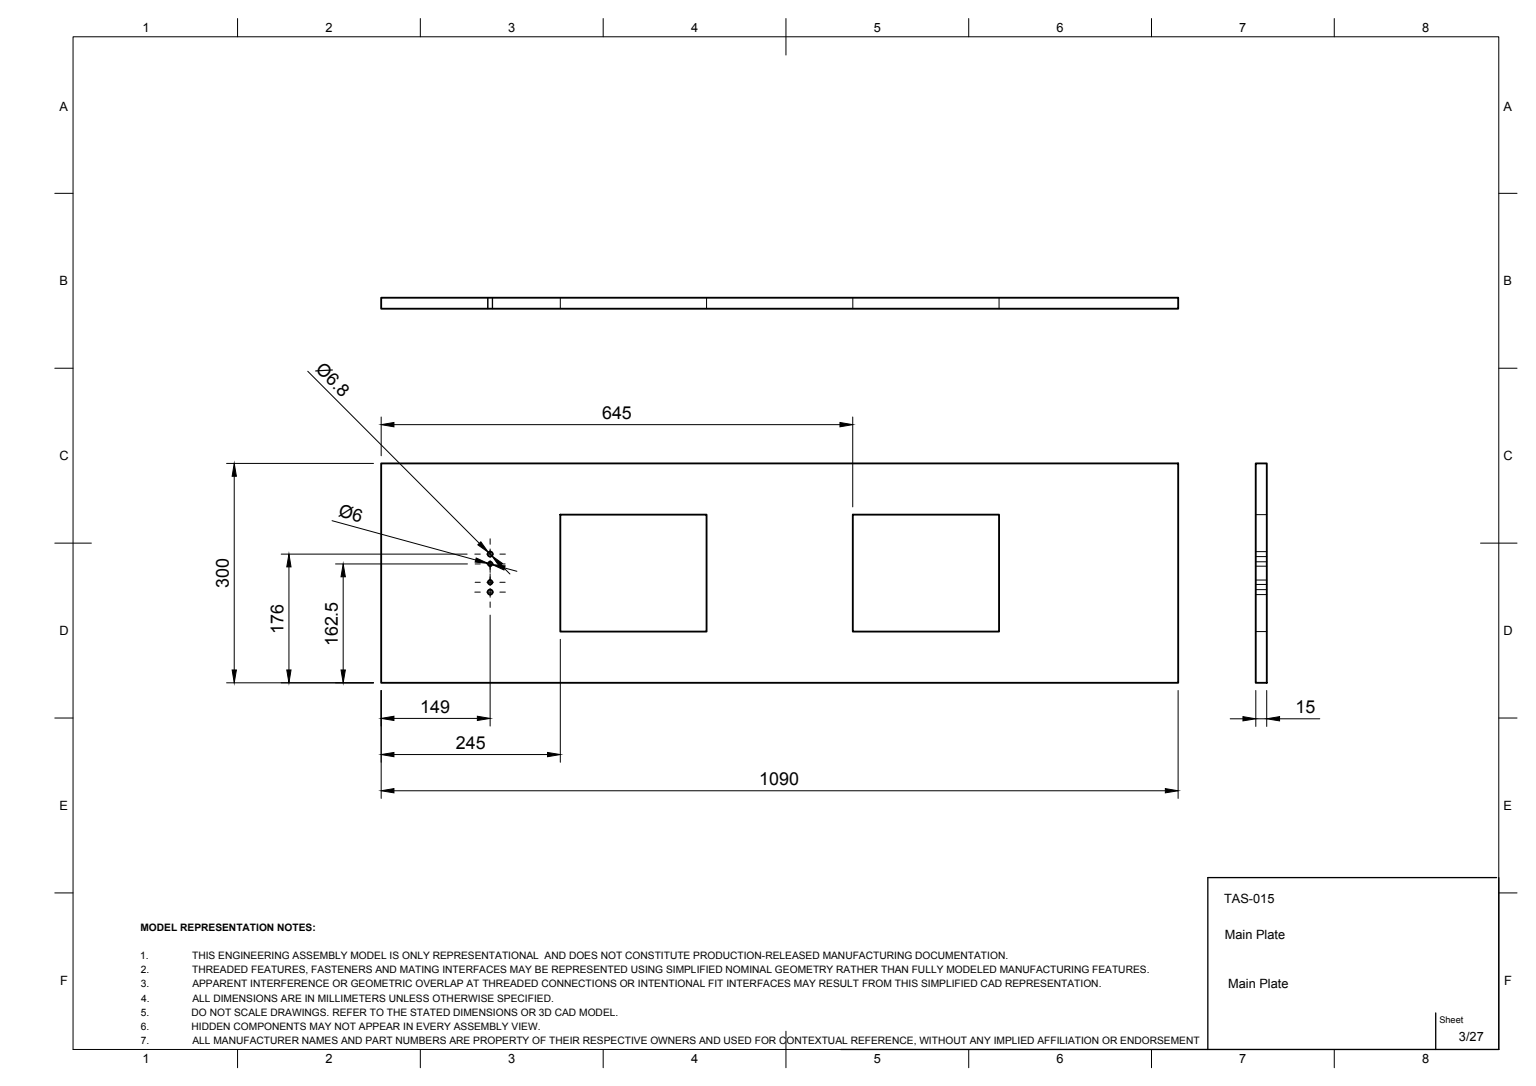
ISO-10303-21;
HEADER;
/* Generated by software containing ST-Developer
 * from STEP Tools, Inc. (www.steptools.com) 
 */

FILE_DESCRIPTION(
/* description */ ('STEP AP214'),
/* implementation_level */ '2;1');

FILE_NAME(
/* name */ 'Main Plate.step',
/* time_stamp */ '2026-11-15T14:49:54-08:00',
/* author */ (''),
/* organization */ (''),
/* preprocessor_version */ 'ST-DEVELOPER v20.2',
/* originating_system */ 'Autodesk Translation Framework v15.17.0.0',
/* authorisation */ '');

FILE_SCHEMA (('AUTOMOTIVE_DESIGN { 1 0 10303 214 3 1 1 }'));
ENDSEC;

DATA;
#10=MECHANICAL_DESIGN_GEOMETRIC_PRESENTATION_REPRESENTATION('',(#1098),#66721);
#1036=SHAPE_REPRESENTATION_RELATIONSHIP('SRR','None',#66891,#1067);
#1067=ADVANCED_BREP_SHAPE_REPRESENTATION('',(#1133),#66682);
#1098=STYLED_ITEM('',(#67095),#1133);
#1133=MANIFOLD_SOLID_BREP('Body1',#25664);
#1168=FACE_BOUND('',#3720,.T.);
#1169=FACE_BOUND('',#3721,.T.);
#1170=FACE_BOUND('',#3722,.T.);
#1171=FACE_BOUND('',#3723,.T.);
#1172=FACE_BOUND('',#3724,.T.);
#1173=FACE_BOUND('',#3725,.T.);
#1174=FACE_BOUND('',#3727,.T.);
#1175=FACE_BOUND('',#3728,.T.);
#1176=FACE_BOUND('',#3729,.T.);
#1177=FACE_BOUND('',#3730,.T.);
#1178=FACE_BOUND('',#3731,.T.);
#1179=FACE_BOUND('',#3732,.T.);
#1498=PLANE('',#26055);
#1499=PLANE('',#26056);
#1500=PLANE('',#26057);
#1501=PLANE('',#26058);
#1502=PLANE('',#26059);
#1503=PLANE('',#26060);
#1504=PLANE('',#26061);
#1505=PLANE('',#26062);
#1506=PLANE('',#26063);
#1507=PLANE('',#26064);
#1508=PLANE('',#26065);
#1509=PLANE('',#26066);
#1510=PLANE('',#26067);
#1511=PLANE('',#26068);
#2269=FACE_OUTER_BOUND('',#3711,.T.);
#2270=FACE_OUTER_BOUND('',#3712,.T.);
#2271=FACE_OUTER_BOUND('',#3713,.T.);
#2272=FACE_OUTER_BOUND('',#3714,.T.);
#2273=FACE_OUTER_BOUND('',#3715,.T.);
#2274=FACE_OUTER_BOUND('',#3716,.T.);
#2275=FACE_OUTER_BOUND('',#3717,.T.);
#2276=FACE_OUTER_BOUND('',#3718,.T.);
#2277=FACE_OUTER_BOUND('',#3719,.T.);
#2278=FACE_OUTER_BOUND('',#3726,.T.);
#2279=FACE_OUTER_BOUND('',#3733,.T.);
#2280=FACE_OUTER_BOUND('',#3734,.T.);
#2281=FACE_OUTER_BOUND('',#3735,.T.);
#2282=FACE_OUTER_BOUND('',#3736,.T.);
#2283=FACE_OUTER_BOUND('',#3737,.T.);
#2284=FACE_OUTER_BOUND('',#3738,.T.);
#2285=FACE_OUTER_BOUND('',#3739,.T.);
#2286=FACE_OUTER_BOUND('',#3740,.T.);
#3711=EDGE_LOOP('',(#16594,#16595,#16596,#16597));
#3712=EDGE_LOOP('',(#16598,#16599,#16600,#16601));
#3713=EDGE_LOOP('',(#16602,#16603,#16604,#16605));
#3714=EDGE_LOOP('',(#16606,#16607,#16608,#16609));
#3715=EDGE_LOOP('',(#16610,#16611,#16612,#16613));
#3716=EDGE_LOOP('',(#16614,#16615,#16616,#16617));
#3717=EDGE_LOOP('',(#16618,#16619,#16620,#16621));
#3718=EDGE_LOOP('',(#16622,#16623,#16624,#16625));
#3719=EDGE_LOOP('',(#16626,#16627,#16628,#16629));
#3720=EDGE_LOOP('',(#16630));
#3721=EDGE_LOOP('',(#16631));
#3722=EDGE_LOOP('',(#16632));
#3723=EDGE_LOOP('',(#16633));
#3724=EDGE_LOOP('',(#16634,#16635,#16636,#16637));
#3725=EDGE_LOOP('',(#16638,#16639,#16640,#16641));
#3726=EDGE_LOOP('',(#16642,#16643,#16644,#16645));
#3727=EDGE_LOOP('',(#16646));
#3728=EDGE_LOOP('',(#16647));
#3729=EDGE_LOOP('',(#16648));
#3730=EDGE_LOOP('',(#16649));
#3731=EDGE_LOOP('',(#16650,#16651,#16652,#16653));
#3732=EDGE_LOOP('',(#16654,#16655,#16656,#16657));
#3733=EDGE_LOOP('',(#16658,#16659,#16660,#16661));
#3734=EDGE_LOOP('',(#16662,#16663,#16664,#16665));
#3735=EDGE_LOOP('',(#16666,#16667,#16668,#16669));
#3736=EDGE_LOOP('',(#16670,#16671,#16672,#16673));
#3737=EDGE_LOOP('',(#16674,#16675,#16676,#16677));
#3738=EDGE_LOOP('',(#16678,#16679,#16680,#16681));
#3739=EDGE_LOOP('',(#16682,#16683,#16684,#16685));
#3740=EDGE_LOOP('',(#16686,#16687,#16688,#16689));
#5483=LINE('',#36181,#7472);
#5484=LINE('',#36187,#7473);
#5485=LINE('',#36193,#7474);
#5486=LINE('',#36199,#7475);
#5487=LINE('',#36204,#7476);
#5488=LINE('',#36206,#7477);
#5489=LINE('',#36208,#7478);
#5490=LINE('',#36209,#7479);
#5491=LINE('',#36212,#7480);
#5492=LINE('',#36214,#7481);
#5493=LINE('',#36215,#7482);
#5494=LINE('',#36218,#7483);
#5495=LINE('',#36220,#7484);
#5496=LINE('',#36221,#7485);
#5497=LINE('',#36223,#7486);
#5498=LINE('',#36224,#7487);
#5499=LINE('',#36228,#7488);
#5500=LINE('',#36230,#7489);
#5501=LINE('',#36232,#7490);
#5502=LINE('',#36233,#7491);
#5503=LINE('',#36236,#7492);
#5504=LINE('',#36238,#7493);
#5505=LINE('',#36240,#7494);
#5506=LINE('',#36241,#7495);
#5507=LINE('',#36245,#7496);
#5508=LINE('',#36247,#7497);
#5509=LINE('',#36249,#7498);
#5510=LINE('',#36250,#7499);
#5511=LINE('',#36253,#7500);
#5512=LINE('',#36255,#7501);
#5513=LINE('',#36257,#7502);
#5514=LINE('',#36258,#7503);
#5515=LINE('',#36260,#7504);
#5516=LINE('',#36261,#7505);
#5517=LINE('',#36263,#7506);
#5518=LINE('',#36265,#7507);
#5519=LINE('',#36268,#7508);
#5520=LINE('',#36269,#7509);
#5521=LINE('',#36271,#7510);
#5522=LINE('',#36273,#7511);
#7472=VECTOR('',#28764,3.4);
#7473=VECTOR('',#28771,3.4);
#7474=VECTOR('',#28778,2.99999999999999);
#7475=VECTOR('',#28785,2.99999999999999);
#7476=VECTOR('',#28790,1000.);
#7477=VECTOR('',#28791,1000.);
#7478=VECTOR('',#28792,1000.);
#7479=VECTOR('',#28793,1000.);
#7480=VECTOR('',#28796,1000.);
#7481=VECTOR('',#28797,1000.);
#7482=VECTOR('',#28798,1000.);
#7483=VECTOR('',#28801,1000.);
#7484=VECTOR('',#28802,1000.);
#7485=VECTOR('',#28803,1000.);
#7486=VECTOR('',#28806,1000.);
#7487=VECTOR('',#28807,1000.);
#7488=VECTOR('',#28810,1000.);
#7489=VECTOR('',#28811,1000.);
#7490=VECTOR('',#28812,1000.);
#7491=VECTOR('',#28813,1000.);
#7492=VECTOR('',#28814,1000.);
#7493=VECTOR('',#28815,1000.);
#7494=VECTOR('',#28816,1000.);
#7495=VECTOR('',#28817,1000.);
#7496=VECTOR('',#28820,1000.);
#7497=VECTOR('',#28821,1000.);
#7498=VECTOR('',#28822,1000.);
#7499=VECTOR('',#28823,1000.);
#7500=VECTOR('',#28824,1000.);
#7501=VECTOR('',#28825,1000.);
#7502=VECTOR('',#28826,1000.);
#7503=VECTOR('',#28827,1000.);
#7504=VECTOR('',#28830,1000.);
#7505=VECTOR('',#28831,1000.);
#7506=VECTOR('',#28834,1000.);
#7507=VECTOR('',#28837,1000.);
#7508=VECTOR('',#28842,1000.);
#7509=VECTOR('',#28843,1000.);
#7510=VECTOR('',#28846,1000.);
#7511=VECTOR('',#28849,1000.);
#9461=CIRCLE('',#26044,3.4);
#9462=CIRCLE('',#26045,3.4);
#9463=CIRCLE('',#26047,3.4);
#9464=CIRCLE('',#26048,3.4);
#9465=CIRCLE('',#26050,3.);
#9466=CIRCLE('',#26051,2.99999999999999);
#9467=CIRCLE('',#26053,3.);
#9468=CIRCLE('',#26054,2.99999999999999);
#10638=VERTEX_POINT('',#36178);
#10639=VERTEX_POINT('',#36180);
#10640=VERTEX_POINT('',#36184);
#10641=VERTEX_POINT('',#36186);
#10642=VERTEX_POINT('',#36190);
#10643=VERTEX_POINT('',#36192);
#10644=VERTEX_POINT('',#36196);
#10645=VERTEX_POINT('',#36198);
#10646=VERTEX_POINT('',#36202);
#10647=VERTEX_POINT('',#36203);
#10648=VERTEX_POINT('',#36205);
#10649=VERTEX_POINT('',#36207);
#10650=VERTEX_POINT('',#36211);
#10651=VERTEX_POINT('',#36213);
#10652=VERTEX_POINT('',#36217);
#10653=VERTEX_POINT('',#36219);
#10654=VERTEX_POINT('',#36226);
#10655=VERTEX_POINT('',#36227);
#10656=VERTEX_POINT('',#36229);
#10657=VERTEX_POINT('',#36231);
#10658=VERTEX_POINT('',#36234);
#10659=VERTEX_POINT('',#36235);
#10660=VERTEX_POINT('',#36237);
#10661=VERTEX_POINT('',#36239);
#10662=VERTEX_POINT('',#36243);
#10663=VERTEX_POINT('',#36244);
#10664=VERTEX_POINT('',#36246);
#10665=VERTEX_POINT('',#36248);
#10666=VERTEX_POINT('',#36251);
#10667=VERTEX_POINT('',#36252);
#10668=VERTEX_POINT('',#36254);
#10669=VERTEX_POINT('',#36256);
#12990=EDGE_CURVE('',#10638,#10638,#9461,.T.);
#12991=EDGE_CURVE('',#10638,#10639,#5483,.T.);
#12992=EDGE_CURVE('',#10639,#10639,#9462,.T.);
#12993=EDGE_CURVE('',#10640,#10640,#9463,.T.);
#12994=EDGE_CURVE('',#10640,#10641,#5484,.T.);
#12995=EDGE_CURVE('',#10641,#10641,#9464,.T.);
#12996=EDGE_CURVE('',#10642,#10642,#9465,.T.);
#12997=EDGE_CURVE('',#10642,#10643,#5485,.T.);
#12998=EDGE_CURVE('',#10643,#10643,#9466,.T.);
#12999=EDGE_CURVE('',#10644,#10644,#9467,.T.);
#13000=EDGE_CURVE('',#10644,#10645,#5486,.T.);
#13001=EDGE_CURVE('',#10645,#10645,#9468,.T.);
#13002=EDGE_CURVE('',#10646,#10647,#5487,.T.);
#13003=EDGE_CURVE('',#10648,#10647,#5488,.T.);
#13004=EDGE_CURVE('',#10649,#10648,#5489,.T.);
#13005=EDGE_CURVE('',#10649,#10646,#5490,.T.);
#13006=EDGE_CURVE('',#10647,#10650,#5491,.T.);
#13007=EDGE_CURVE('',#10651,#10650,#5492,.T.);
#13008=EDGE_CURVE('',#10648,#10651,#5493,.T.);
#13009=EDGE_CURVE('',#10650,#10652,#5494,.T.);
#13010=EDGE_CURVE('',#10653,#10652,#5495,.T.);
#13011=EDGE_CURVE('',#10651,#10653,#5496,.T.);
#13012=EDGE_CURVE('',#10652,#10646,#5497,.T.);
#13013=EDGE_CURVE('',#10653,#10649,#5498,.T.);
#13014=EDGE_CURVE('',#10654,#10655,#5499,.T.);
#13015=EDGE_CURVE('',#10656,#10654,#5500,.T.);
#13016=EDGE_CURVE('',#10657,#10656,#5501,.T.);
#13017=EDGE_CURVE('',#10655,#10657,#5502,.T.);
#13018=EDGE_CURVE('',#10658,#10659,#5503,.T.);
#13019=EDGE_CURVE('',#10660,#10658,#5504,.T.);
#13020=EDGE_CURVE('',#10661,#10660,#5505,.T.);
#13021=EDGE_CURVE('',#10659,#10661,#5506,.T.);
#13022=EDGE_CURVE('',#10662,#10663,#5507,.T.);
#13023=EDGE_CURVE('',#10663,#10664,#5508,.T.);
#13024=EDGE_CURVE('',#10664,#10665,#5509,.T.);
#13025=EDGE_CURVE('',#10665,#10662,#5510,.T.);
#13026=EDGE_CURVE('',#10666,#10667,#5511,.T.);
#13027=EDGE_CURVE('',#10667,#10668,#5512,.T.);
#13028=EDGE_CURVE('',#10668,#10669,#5513,.T.);
#13029=EDGE_CURVE('',#10669,#10666,#5514,.T.);
#13030=EDGE_CURVE('',#10667,#10658,#5515,.T.);
#13031=EDGE_CURVE('',#10666,#10660,#5516,.T.);
#13032=EDGE_CURVE('',#10669,#10661,#5517,.T.);
#13033=EDGE_CURVE('',#10668,#10659,#5518,.T.);
#13034=EDGE_CURVE('',#10663,#10654,#5519,.T.);
#13035=EDGE_CURVE('',#10662,#10656,#5520,.T.);
#13036=EDGE_CURVE('',#10665,#10657,#5521,.T.);
#13037=EDGE_CURVE('',#10664,#10655,#5522,.T.);
#16594=ORIENTED_EDGE('',*,*,#12990,.F.);
#16595=ORIENTED_EDGE('',*,*,#12991,.T.);
#16596=ORIENTED_EDGE('',*,*,#12992,.T.);
#16597=ORIENTED_EDGE('',*,*,#12991,.F.);
#16598=ORIENTED_EDGE('',*,*,#12993,.F.);
#16599=ORIENTED_EDGE('',*,*,#12994,.T.);
#16600=ORIENTED_EDGE('',*,*,#12995,.T.);
#16601=ORIENTED_EDGE('',*,*,#12994,.F.);
#16602=ORIENTED_EDGE('',*,*,#12996,.F.);
#16603=ORIENTED_EDGE('',*,*,#12997,.T.);
#16604=ORIENTED_EDGE('',*,*,#12998,.T.);
#16605=ORIENTED_EDGE('',*,*,#12997,.F.);
#16606=ORIENTED_EDGE('',*,*,#12999,.F.);
#16607=ORIENTED_EDGE('',*,*,#13000,.T.);
#16608=ORIENTED_EDGE('',*,*,#13001,.T.);
#16609=ORIENTED_EDGE('',*,*,#13000,.F.);
#16610=ORIENTED_EDGE('',*,*,#13002,.T.);
#16611=ORIENTED_EDGE('',*,*,#13003,.F.);
#16612=ORIENTED_EDGE('',*,*,#13004,.F.);
#16613=ORIENTED_EDGE('',*,*,#13005,.T.);
#16614=ORIENTED_EDGE('',*,*,#13006,.T.);
#16615=ORIENTED_EDGE('',*,*,#13007,.F.);
#16616=ORIENTED_EDGE('',*,*,#13008,.F.);
#16617=ORIENTED_EDGE('',*,*,#13003,.T.);
#16618=ORIENTED_EDGE('',*,*,#13009,.T.);
#16619=ORIENTED_EDGE('',*,*,#13010,.F.);
#16620=ORIENTED_EDGE('',*,*,#13011,.F.);
#16621=ORIENTED_EDGE('',*,*,#13007,.T.);
#16622=ORIENTED_EDGE('',*,*,#13012,.T.);
#16623=ORIENTED_EDGE('',*,*,#13005,.F.);
#16624=ORIENTED_EDGE('',*,*,#13013,.F.);
#16625=ORIENTED_EDGE('',*,*,#13010,.T.);
#16626=ORIENTED_EDGE('',*,*,#13004,.T.);
#16627=ORIENTED_EDGE('',*,*,#13008,.T.);
#16628=ORIENTED_EDGE('',*,*,#13011,.T.);
#16629=ORIENTED_EDGE('',*,*,#13013,.T.);
#16630=ORIENTED_EDGE('',*,*,#12992,.F.);
#16631=ORIENTED_EDGE('',*,*,#12995,.F.);
#16632=ORIENTED_EDGE('',*,*,#12998,.F.);
#16633=ORIENTED_EDGE('',*,*,#13001,.F.);
#16634=ORIENTED_EDGE('',*,*,#13014,.F.);
#16635=ORIENTED_EDGE('',*,*,#13015,.F.);
#16636=ORIENTED_EDGE('',*,*,#13016,.F.);
#16637=ORIENTED_EDGE('',*,*,#13017,.F.);
#16638=ORIENTED_EDGE('',*,*,#13018,.F.);
#16639=ORIENTED_EDGE('',*,*,#13019,.F.);
#16640=ORIENTED_EDGE('',*,*,#13020,.F.);
#16641=ORIENTED_EDGE('',*,*,#13021,.F.);
#16642=ORIENTED_EDGE('',*,*,#13002,.F.);
#16643=ORIENTED_EDGE('',*,*,#13012,.F.);
#16644=ORIENTED_EDGE('',*,*,#13009,.F.);
#16645=ORIENTED_EDGE('',*,*,#13006,.F.);
#16646=ORIENTED_EDGE('',*,*,#12990,.T.);
#16647=ORIENTED_EDGE('',*,*,#12993,.T.);
#16648=ORIENTED_EDGE('',*,*,#12996,.T.);
#16649=ORIENTED_EDGE('',*,*,#12999,.T.);
#16650=ORIENTED_EDGE('',*,*,#13022,.T.);
#16651=ORIENTED_EDGE('',*,*,#13023,.T.);
#16652=ORIENTED_EDGE('',*,*,#13024,.T.);
#16653=ORIENTED_EDGE('',*,*,#13025,.T.);
#16654=ORIENTED_EDGE('',*,*,#13026,.T.);
#16655=ORIENTED_EDGE('',*,*,#13027,.T.);
#16656=ORIENTED_EDGE('',*,*,#13028,.T.);
#16657=ORIENTED_EDGE('',*,*,#13029,.T.);
#16658=ORIENTED_EDGE('',*,*,#13019,.T.);
#16659=ORIENTED_EDGE('',*,*,#13030,.F.);
#16660=ORIENTED_EDGE('',*,*,#13026,.F.);
#16661=ORIENTED_EDGE('',*,*,#13031,.T.);
#16662=ORIENTED_EDGE('',*,*,#13020,.T.);
#16663=ORIENTED_EDGE('',*,*,#13031,.F.);
#16664=ORIENTED_EDGE('',*,*,#13029,.F.);
#16665=ORIENTED_EDGE('',*,*,#13032,.T.);
#16666=ORIENTED_EDGE('',*,*,#13021,.T.);
#16667=ORIENTED_EDGE('',*,*,#13032,.F.);
#16668=ORIENTED_EDGE('',*,*,#13028,.F.);
#16669=ORIENTED_EDGE('',*,*,#13033,.T.);
#16670=ORIENTED_EDGE('',*,*,#13018,.T.);
#16671=ORIENTED_EDGE('',*,*,#13033,.F.);
#16672=ORIENTED_EDGE('',*,*,#13027,.F.);
#16673=ORIENTED_EDGE('',*,*,#13030,.T.);
#16674=ORIENTED_EDGE('',*,*,#13015,.T.);
#16675=ORIENTED_EDGE('',*,*,#13034,.F.);
#16676=ORIENTED_EDGE('',*,*,#13022,.F.);
#16677=ORIENTED_EDGE('',*,*,#13035,.T.);
#16678=ORIENTED_EDGE('',*,*,#13016,.T.);
#16679=ORIENTED_EDGE('',*,*,#13035,.F.);
#16680=ORIENTED_EDGE('',*,*,#13025,.F.);
#16681=ORIENTED_EDGE('',*,*,#13036,.T.);
#16682=ORIENTED_EDGE('',*,*,#13017,.T.);
#16683=ORIENTED_EDGE('',*,*,#13036,.F.);
#16684=ORIENTED_EDGE('',*,*,#13024,.F.);
#16685=ORIENTED_EDGE('',*,*,#13037,.T.);
#16686=ORIENTED_EDGE('',*,*,#13014,.T.);
#16687=ORIENTED_EDGE('',*,*,#13037,.F.);
#16688=ORIENTED_EDGE('',*,*,#13023,.F.);
#16689=ORIENTED_EDGE('',*,*,#13034,.T.);
#23802=CYLINDRICAL_SURFACE('',#26043,3.4);
#23803=CYLINDRICAL_SURFACE('',#26046,3.4);
#23804=CYLINDRICAL_SURFACE('',#26049,2.99999999999999);
#23805=CYLINDRICAL_SURFACE('',#26052,2.99999999999999);
#24222=ADVANCED_FACE('',(#2269),#23802,.F.);
#24223=ADVANCED_FACE('',(#2270),#23803,.F.);
#24224=ADVANCED_FACE('',(#2271),#23804,.F.);
#24225=ADVANCED_FACE('',(#2272),#23805,.F.);
#24226=ADVANCED_FACE('',(#2273),#1498,.F.);
#24227=ADVANCED_FACE('',(#2274),#1499,.F.);
#24228=ADVANCED_FACE('',(#2275),#1500,.F.);
#24229=ADVANCED_FACE('',(#2276),#1501,.F.);
#24230=ADVANCED_FACE('',(#2277,#1168,#1169,#1170,#1171,#1172,#1173),#1502,
 .F.);
#24231=ADVANCED_FACE('',(#2278,#1174,#1175,#1176,#1177,#1178,#1179),#1503,
 .T.);
#24232=ADVANCED_FACE('',(#2279),#1504,.F.);
#24233=ADVANCED_FACE('',(#2280),#1505,.F.);
#24234=ADVANCED_FACE('',(#2281),#1506,.F.);
#24235=ADVANCED_FACE('',(#2282),#1507,.F.);
#24236=ADVANCED_FACE('',(#2283),#1508,.F.);
#24237=ADVANCED_FACE('',(#2284),#1509,.F.);
#24238=ADVANCED_FACE('',(#2285),#1510,.F.);
#24239=ADVANCED_FACE('',(#2286),#1511,.F.);
#25664=CLOSED_SHELL('',(#24222,#24223,#24224,#24225,#24226,#24227,#24228,
#24229,#24230,#24231,#24232,#24233,#24234,#24235,#24236,#24237,#24238,#24239));
#26042=AXIS2_PLACEMENT_3D('',#36176,#28758,#28759);
#26043=AXIS2_PLACEMENT_3D('',#36177,#28760,#28761);
#26044=AXIS2_PLACEMENT_3D('',#36179,#28762,#28763);
#26045=AXIS2_PLACEMENT_3D('',#36182,#28765,#28766);
#26046=AXIS2_PLACEMENT_3D('',#36183,#28767,#28768);
#26047=AXIS2_PLACEMENT_3D('',#36185,#28769,#28770);
#26048=AXIS2_PLACEMENT_3D('',#36188,#28772,#28773);
#26049=AXIS2_PLACEMENT_3D('',#36189,#28774,#28775);
#26050=AXIS2_PLACEMENT_3D('',#36191,#28776,#28777);
#26051=AXIS2_PLACEMENT_3D('',#36194,#28779,#28780);
#26052=AXIS2_PLACEMENT_3D('',#36195,#28781,#28782);
#26053=AXIS2_PLACEMENT_3D('',#36197,#28783,#28784);
#26054=AXIS2_PLACEMENT_3D('',#36200,#28786,#28787);
#26055=AXIS2_PLACEMENT_3D('',#36201,#28788,#28789);
#26056=AXIS2_PLACEMENT_3D('',#36210,#28794,#28795);
#26057=AXIS2_PLACEMENT_3D('',#36216,#28799,#28800);
#26058=AXIS2_PLACEMENT_3D('',#36222,#28804,#28805);
#26059=AXIS2_PLACEMENT_3D('',#36225,#28808,#28809);
#26060=AXIS2_PLACEMENT_3D('',#36242,#28818,#28819);
#26061=AXIS2_PLACEMENT_3D('',#36259,#28828,#28829);
#26062=AXIS2_PLACEMENT_3D('',#36262,#28832,#28833);
#26063=AXIS2_PLACEMENT_3D('',#36264,#28835,#28836);
#26064=AXIS2_PLACEMENT_3D('',#36266,#28838,#28839);
#26065=AXIS2_PLACEMENT_3D('',#36267,#28840,#28841);
#26066=AXIS2_PLACEMENT_3D('',#36270,#28844,#28845);
#26067=AXIS2_PLACEMENT_3D('',#36272,#28847,#28848);
#26068=AXIS2_PLACEMENT_3D('',#36274,#28850,#28851);
#28758=DIRECTION('axis',(0.,0.,1.));
#28759=DIRECTION('refdir',(1.,0.,0.));
#28760=DIRECTION('center_axis',(0.,0.,1.));
#28761=DIRECTION('ref_axis',(1.,0.,0.));
#28762=DIRECTION('center_axis',(0.,0.,1.));
#28763=DIRECTION('ref_axis',(1.,0.,0.));
#28764=DIRECTION('',(0.,0.,1.));
#28765=DIRECTION('center_axis',(0.,0.,1.));
#28766=DIRECTION('ref_axis',(1.,0.,0.));
#28767=DIRECTION('center_axis',(0.,0.,1.));
#28768=DIRECTION('ref_axis',(1.,0.,0.));
#28769=DIRECTION('center_axis',(0.,0.,1.));
#28770=DIRECTION('ref_axis',(1.,0.,0.));
#28771=DIRECTION('',(0.,0.,1.));
#28772=DIRECTION('center_axis',(0.,0.,1.));
#28773=DIRECTION('ref_axis',(1.,0.,0.));
#28774=DIRECTION('center_axis',(0.,0.,1.));
#28775=DIRECTION('ref_axis',(1.,0.,0.));
#28776=DIRECTION('center_axis',(0.,0.,1.));
#28777=DIRECTION('ref_axis',(1.,0.,0.));
#28778=DIRECTION('',(0.,0.,1.));
#28779=DIRECTION('center_axis',(0.,0.,1.));
#28780=DIRECTION('ref_axis',(1.,0.,0.));
#28781=DIRECTION('center_axis',(0.,0.,1.));
#28782=DIRECTION('ref_axis',(1.,0.,0.));
#28783=DIRECTION('center_axis',(0.,0.,1.));
#28784=DIRECTION('ref_axis',(1.,0.,0.));
#28785=DIRECTION('',(0.,0.,1.));
#28786=DIRECTION('center_axis',(0.,0.,1.));
#28787=DIRECTION('ref_axis',(1.,0.,0.));
#28788=DIRECTION('center_axis',(-1.,0.,0.));
#28789=DIRECTION('ref_axis',(0.,0.,1.));
#28790=DIRECTION('',(0.,1.,0.));
#28791=DIRECTION('',(0.,0.,-1.));
#28792=DIRECTION('',(0.,1.,0.));
#28793=DIRECTION('',(0.,0.,-1.));
#28794=DIRECTION('center_axis',(0.,-1.,0.));
#28795=DIRECTION('ref_axis',(0.,0.,-1.));
#28796=DIRECTION('',(-1.,0.,0.));
#28797=DIRECTION('',(0.,0.,-1.));
#28798=DIRECTION('',(-1.,0.,0.));
#28799=DIRECTION('center_axis',(1.,0.,0.));
#28800=DIRECTION('ref_axis',(0.,0.,-1.));
#28801=DIRECTION('',(0.,-1.,0.));
#28802=DIRECTION('',(0.,0.,-1.));
#28803=DIRECTION('',(0.,-1.,0.));
#28804=DIRECTION('center_axis',(0.,1.,0.));
#28805=DIRECTION('ref_axis',(0.,0.,1.));
#28806=DIRECTION('',(1.,0.,0.));
#28807=DIRECTION('',(1.,0.,0.));
#28808=DIRECTION('center_axis',(0.,0.,-1.));
#28809=DIRECTION('ref_axis',(-1.,0.,0.));
#28810=DIRECTION('',(1.,-3.46944695195361E-16,0.));
#28811=DIRECTION('',(6.93889390390723E-17,-1.,0.));
#28812=DIRECTION('',(-1.,0.,0.));
#28813=DIRECTION('',(-1.38777878078145E-16,1.,0.));
#28814=DIRECTION('',(1.,0.,0.));
#28815=DIRECTION('',(1.38777878078145E-16,-1.,0.));
#28816=DIRECTION('',(-1.,0.,0.));
#28817=DIRECTION('',(-2.77555756156289E-16,1.,0.));
#28818=DIRECTION('center_axis',(0.,0.,-1.));
#28819=DIRECTION('ref_axis',(-1.,0.,0.));
#28820=DIRECTION('',(6.93889390390723E-17,-1.,0.));
#28821=DIRECTION('',(1.,-3.46944695195361E-16,0.));
#28822=DIRECTION('',(-1.38777878078145E-16,1.,0.));
#28823=DIRECTION('',(-1.,0.,0.));
#28824=DIRECTION('',(1.38777878078145E-16,-1.,0.));
#28825=DIRECTION('',(1.,0.,0.));
#28826=DIRECTION('',(-2.77555756156289E-16,1.,0.));
#28827=DIRECTION('',(-1.,0.,0.));
#28828=DIRECTION('center_axis',(-1.,-1.38777878078145E-16,0.));
#28829=DIRECTION('ref_axis',(1.38777878078145E-16,-1.,0.));
#28830=DIRECTION('',(0.,0.,1.));
#28831=DIRECTION('',(0.,0.,1.));
#28832=DIRECTION('center_axis',(0.,1.,0.));
#28833=DIRECTION('ref_axis',(0.,0.,1.));
#28834=DIRECTION('',(0.,0.,1.));
#28835=DIRECTION('center_axis',(1.,2.77555756156289E-16,0.));
#28836=DIRECTION('ref_axis',(-2.77555756156289E-16,1.,0.));
#28837=DIRECTION('',(0.,0.,1.));
#28838=DIRECTION('center_axis',(0.,-1.,0.));
#28839=DIRECTION('ref_axis',(0.,0.,-1.));
#28840=DIRECTION('center_axis',(-1.,-6.93889390390723E-17,0.));
#28841=DIRECTION('ref_axis',(6.93889390390723E-17,-1.,0.));
#28842=DIRECTION('',(0.,0.,1.));
#28843=DIRECTION('',(0.,0.,1.));
#28844=DIRECTION('center_axis',(0.,1.,0.));
#28845=DIRECTION('ref_axis',(0.,0.,1.));
#28846=DIRECTION('',(0.,0.,1.));
#28847=DIRECTION('center_axis',(1.,1.38777878078145E-16,0.));
#28848=DIRECTION('ref_axis',(-1.38777878078145E-16,1.,0.));
#28849=DIRECTION('',(0.,0.,1.));
#28850=DIRECTION('center_axis',(-3.46944695195361E-16,-1.,0.));
#28851=DIRECTION('ref_axis',(1.,-3.46944695195361E-16,0.));
#36176=CARTESIAN_POINT('',(0.,0.,0.));
#36177=CARTESIAN_POINT('Origin',(-26.,396.,7.5));
#36178=CARTESIAN_POINT('',(-29.4,396.,-7.5));
#36179=CARTESIAN_POINT('Origin',(-26.,396.,-7.5));
#36180=CARTESIAN_POINT('',(-29.4,396.,7.5));
#36181=CARTESIAN_POINT('',(-29.4,396.,7.5));
#36182=CARTESIAN_POINT('Origin',(-26.,396.,7.5));
#36183=CARTESIAN_POINT('Origin',(26.,396.,7.5));
#36184=CARTESIAN_POINT('',(22.6,396.,-7.5));
#36185=CARTESIAN_POINT('Origin',(26.,396.,-7.5));
#36186=CARTESIAN_POINT('',(22.6,396.,7.5));
#36187=CARTESIAN_POINT('',(22.6,396.,7.5));
#36188=CARTESIAN_POINT('Origin',(26.,396.,7.5));
#36189=CARTESIAN_POINT('Origin',(-12.5,396.,7.5));
#36190=CARTESIAN_POINT('',(-15.5,396.,-7.5));
#36191=CARTESIAN_POINT('Origin',(-12.5,396.,-7.5));
#36192=CARTESIAN_POINT('',(-15.5,396.,7.5));
#36193=CARTESIAN_POINT('',(-15.5,396.,7.5));
#36194=CARTESIAN_POINT('Origin',(-12.5,396.,7.5));
#36195=CARTESIAN_POINT('Origin',(12.5,396.,7.5));
#36196=CARTESIAN_POINT('',(9.50000000000001,396.,-7.5));
#36197=CARTESIAN_POINT('Origin',(12.5,396.,-7.5));
#36198=CARTESIAN_POINT('',(9.50000000000001,396.,7.5));
#36199=CARTESIAN_POINT('',(9.50000000000001,396.,7.5));
#36200=CARTESIAN_POINT('Origin',(12.5,396.,7.5));
#36201=CARTESIAN_POINT('Origin',(150.,-545.,7.5));
#36202=CARTESIAN_POINT('',(150.,-545.,-7.5));
#36203=CARTESIAN_POINT('',(150.,545.,-7.5));
#36204=CARTESIAN_POINT('',(150.,-545.,-7.5));
#36205=CARTESIAN_POINT('',(150.,545.,7.5));
#36206=CARTESIAN_POINT('',(150.,545.,7.5));
#36207=CARTESIAN_POINT('',(150.,-545.,7.5));
#36208=CARTESIAN_POINT('',(150.,-545.,7.5));
#36209=CARTESIAN_POINT('',(150.,-545.,7.5));
#36210=CARTESIAN_POINT('Origin',(-150.,545.,7.5));
#36211=CARTESIAN_POINT('',(-150.,545.,-7.5));
#36212=CARTESIAN_POINT('',(-150.,545.,-7.5));
#36213=CARTESIAN_POINT('',(-150.,545.,7.5));
#36214=CARTESIAN_POINT('',(-150.,545.,7.5));
#36215=CARTESIAN_POINT('',(-150.,545.,7.5));
#36216=CARTESIAN_POINT('Origin',(-150.,-545.,7.5));
#36217=CARTESIAN_POINT('',(-150.,-545.,-7.5));
#36218=CARTESIAN_POINT('',(-150.,-545.,-7.5));
#36219=CARTESIAN_POINT('',(-150.,-545.,7.5));
#36220=CARTESIAN_POINT('',(-150.,-545.,7.5));
#36221=CARTESIAN_POINT('',(-150.,-545.,7.5));
#36222=CARTESIAN_POINT('Origin',(-150.,-545.,7.5));
#36223=CARTESIAN_POINT('',(-150.,-545.,-7.5));
#36224=CARTESIAN_POINT('',(-150.,-545.,7.5));
#36225=CARTESIAN_POINT('Origin',(0.,0.,7.5));
#36226=CARTESIAN_POINT('',(-80.,-300.,7.5));
#36227=CARTESIAN_POINT('',(80.,-300.,7.5));
#36228=CARTESIAN_POINT('',(-80.,-300.,7.5));
#36229=CARTESIAN_POINT('',(-80.,-100.,7.5));
#36230=CARTESIAN_POINT('',(-80.,-100.,7.5));
#36231=CARTESIAN_POINT('',(80.,-100.,7.5));
#36232=CARTESIAN_POINT('',(-80.,-100.,7.5));
#36233=CARTESIAN_POINT('',(80.,-100.,7.5));
#36234=CARTESIAN_POINT('',(-80.,99.9999999999999,7.5));
#36235=CARTESIAN_POINT('',(80.,99.9999999999999,7.5));
#36236=CARTESIAN_POINT('',(-80.,99.9999999999999,7.5));
#36237=CARTESIAN_POINT('',(-80.0000000000001,300.,7.5));
#36238=CARTESIAN_POINT('',(-80.0000000000001,300.,7.5));
#36239=CARTESIAN_POINT('',(79.9999999999999,300.,7.5));
#36240=CARTESIAN_POINT('',(-80.0000000000001,300.,7.5));
#36241=CARTESIAN_POINT('',(79.9999999999999,300.,7.5));
#36242=CARTESIAN_POINT('Origin',(0.,0.,-7.5));
#36243=CARTESIAN_POINT('',(-80.,-100.,-7.5));
#36244=CARTESIAN_POINT('',(-80.,-300.,-7.5));
#36245=CARTESIAN_POINT('',(-80.,-100.,-7.5));
#36246=CARTESIAN_POINT('',(80.,-300.,-7.5));
#36247=CARTESIAN_POINT('',(-80.,-300.,-7.5));
#36248=CARTESIAN_POINT('',(80.,-100.,-7.5));
#36249=CARTESIAN_POINT('',(80.,-100.,-7.5));
#36250=CARTESIAN_POINT('',(-80.,-100.,-7.5));
#36251=CARTESIAN_POINT('',(-80.0000000000001,300.,-7.5));
#36252=CARTESIAN_POINT('',(-80.,99.9999999999999,-7.5));
#36253=CARTESIAN_POINT('',(-80.0000000000001,300.,-7.5));
#36254=CARTESIAN_POINT('',(80.,99.9999999999999,-7.5));
#36255=CARTESIAN_POINT('',(-80.,99.9999999999999,-7.5));
#36256=CARTESIAN_POINT('',(79.9999999999999,300.,-7.5));
#36257=CARTESIAN_POINT('',(79.9999999999999,300.,-7.5));
#36258=CARTESIAN_POINT('',(-80.0000000000001,300.,-7.5));
#36259=CARTESIAN_POINT('Origin',(-80.0000000000001,300.,-7.5));
#36260=CARTESIAN_POINT('',(-80.,99.9999999999999,-7.5));
#36261=CARTESIAN_POINT('',(-80.0000000000001,300.,-7.5));
#36262=CARTESIAN_POINT('Origin',(-80.0000000000001,300.,-7.5));
#36263=CARTESIAN_POINT('',(79.9999999999999,300.,-7.5));
#36264=CARTESIAN_POINT('Origin',(79.9999999999999,300.,-7.5));
#36265=CARTESIAN_POINT('',(80.,99.9999999999999,-7.5));
#36266=CARTESIAN_POINT('Origin',(-80.,99.9999999999999,-7.5));
#36267=CARTESIAN_POINT('Origin',(-80.,-100.,-7.5));
#36268=CARTESIAN_POINT('',(-80.,-300.,-7.5));
#36269=CARTESIAN_POINT('',(-80.,-100.,-7.5));
#36270=CARTESIAN_POINT('Origin',(-80.,-100.,-7.5));
#36271=CARTESIAN_POINT('',(80.,-100.,-7.5));
#36272=CARTESIAN_POINT('Origin',(80.,-100.,-7.5));
#36273=CARTESIAN_POINT('',(80.,-300.,-7.5));
#36274=CARTESIAN_POINT('Origin',(-80.,-300.,-7.5));
#66641=UNCERTAINTY_MEASURE_WITH_UNIT(LENGTH_MEASURE(0.01),#66722,
'DISTANCE_ACCURACY_VALUE',
'Maximum model space distance between geometric entities at asserted c
onnectivities');
#66680=UNCERTAINTY_MEASURE_WITH_UNIT(LENGTH_MEASURE(0.01),#66722,
'DISTANCE_ACCURACY_VALUE',
'Maximum model space distance between geometric entities at asserted c
onnectivities');
#66682=(
GEOMETRIC_REPRESENTATION_CONTEXT(3)
GLOBAL_UNCERTAINTY_ASSIGNED_CONTEXT((#66641))
GLOBAL_UNIT_ASSIGNED_CONTEXT((#66722,#66724,#66725))
REPRESENTATION_CONTEXT('','3D')
);
#66721=(
GEOMETRIC_REPRESENTATION_CONTEXT(3)
GLOBAL_UNCERTAINTY_ASSIGNED_CONTEXT((#66680))
GLOBAL_UNIT_ASSIGNED_CONTEXT((#66722,#66724,#66725))
REPRESENTATION_CONTEXT('','3D')
);
#66722=(
LENGTH_UNIT()
NAMED_UNIT(*)
SI_UNIT(.MILLI.,.METRE.)
);
#66724=(
NAMED_UNIT(*)
PLANE_ANGLE_UNIT()
SI_UNIT($,.RADIAN.)
);
#66725=(
NAMED_UNIT(*)
SI_UNIT($,.STERADIAN.)
SOLID_ANGLE_UNIT()
);
#66727=SHAPE_DEFINITION_REPRESENTATION(#66767,#66891);
#66767=PRODUCT_DEFINITION_SHAPE('',$,#66932);
#66891=SHAPE_REPRESENTATION('',(#26042),#66682);
#66930=PRODUCT_DEFINITION_CONTEXT('part definition',#67052,'design');
#66932=PRODUCT_DEFINITION('Main Plate','Main Plate',#66972,#66930);
#66972=PRODUCT_DEFINITION_FORMATION('',$,#67055);
#67052=APPLICATION_CONTEXT(
'Core Data for Automotive Mechanical Design Process');
#67053=PRODUCT_CONTEXT('part definition',#67052,'mechanical');
#67055=PRODUCT('Main Plate','Main Plate',$,(#67053));
#67095=PRESENTATION_STYLE_ASSIGNMENT((#67097));
#67097=SURFACE_STYLE_USAGE(.BOTH.,#67099);
#67099=SURFACE_SIDE_STYLE('',(#67101));
#67101=SURFACE_STYLE_FILL_AREA(#67103);
#67103=FILL_AREA_STYLE('Opaque(202,209,238)',(#67105));
#67105=FILL_AREA_STYLE_COLOUR('Opaque(202,209,238)',#67107);
#67107=COLOUR_RGB('Opaque(202,209,238)',0.792156862745098,0.819607843137255,
0.933333333333333);
ENDSEC;
END-ISO-10303-21;
